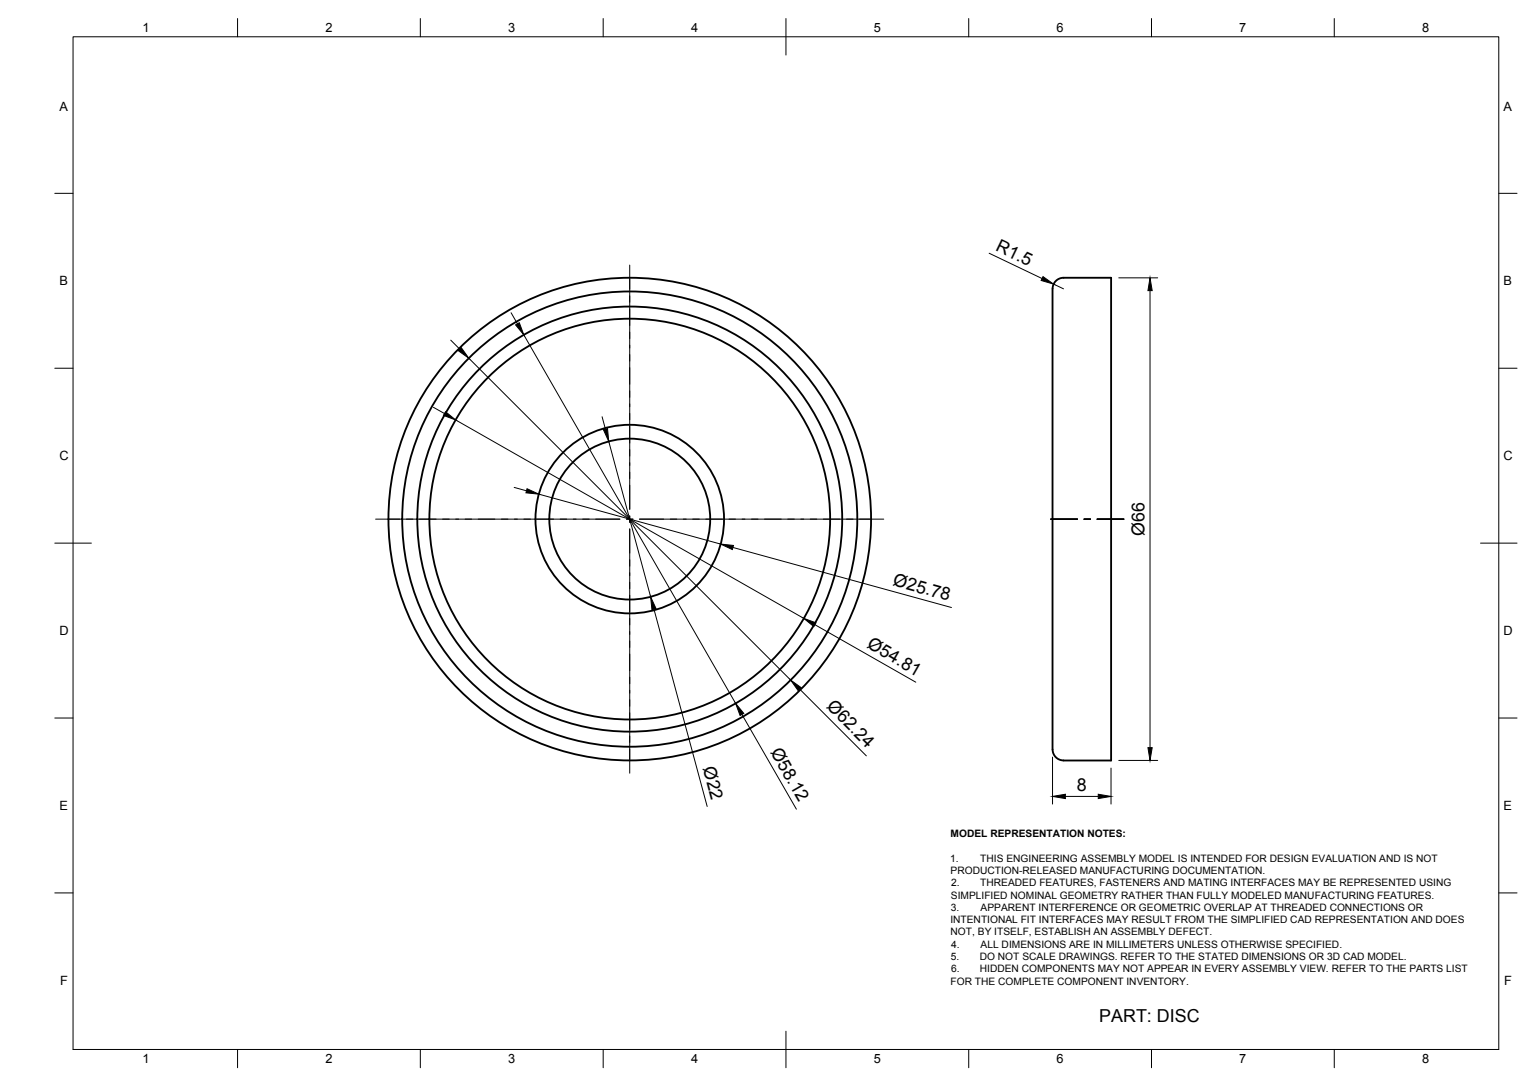
ISO-10303-21;
HEADER;
/* Generated by software containing ST-Developer
 * from STEP Tools, Inc. (www.steptools.com) 
 */

FILE_DESCRIPTION(
/* description */ (''),
/* implementation_level */ '2;1');

FILE_NAME(
/* name */ 'Disc.step',
/* time_stamp */ '2026-10-04T22:47:03-07:00',
/* author */ (''),
/* organization */ (''),
/* preprocessor_version */ 'ST-DEVELOPER v20.2',
/* originating_system */ 'Autodesk Translation Framework v15.15.0.0',
/* authorisation */ '');

FILE_SCHEMA (('AUTOMOTIVE_DESIGN { 1 0 10303 214 3 1 1 }'));
ENDSEC;

DATA;
#10=MECHANICAL_DESIGN_GEOMETRIC_PRESENTATION_REPRESENTATION('',(#81),#19878);
#46=TOROIDAL_SURFACE('',#5269,18.2498324643894,1.5);
#47=TOROIDAL_SURFACE('',#5277,28.1934256722844,1.5);
#48=TOROIDAL_SURFACE('',#5285,31.5,1.5);
#49=TOROIDAL_SURFACE('',#5293,12.,1.);
#67=SHAPE_REPRESENTATION_RELATIONSHIP('SRR','None',#19911,#74);
#74=ADVANCED_BREP_SHAPE_REPRESENTATION('',(#88),#19875);
#81=STYLED_ITEM('',(#19954),#88);
#88=MANIFOLD_SOLID_BREP('Body1',#4829);
#97=FACE_BOUND('',#819,.T.);
#98=FACE_BOUND('',#822,.T.);
#99=FACE_BOUND('',#827,.T.);
#100=FACE_BOUND('',#831,.T.);
#101=FACE_BOUND('',#834,.T.);
#102=FACE_BOUND('',#837,.T.);
#103=FACE_BOUND('',#840,.T.);
#305=PLANE('',#5275);
#306=PLANE('',#5281);
#307=PLANE('',#5290);
#308=PLANE('',#5296);
#309=PLANE('',#5300);
#310=PLANE('',#5304);
#311=PLANE('',#5308);
#534=FACE_OUTER_BOUND('',#816,.T.);
#535=FACE_OUTER_BOUND('',#817,.T.);
#536=FACE_OUTER_BOUND('',#818,.T.);
#537=FACE_OUTER_BOUND('',#820,.T.);
#538=FACE_OUTER_BOUND('',#821,.T.);
#539=FACE_OUTER_BOUND('',#823,.T.);
#540=FACE_OUTER_BOUND('',#824,.T.);
#541=FACE_OUTER_BOUND('',#825,.T.);
#542=FACE_OUTER_BOUND('',#826,.T.);
#543=FACE_OUTER_BOUND('',#828,.T.);
#544=FACE_OUTER_BOUND('',#829,.T.);
#545=FACE_OUTER_BOUND('',#830,.T.);
#546=FACE_OUTER_BOUND('',#832,.T.);
#547=FACE_OUTER_BOUND('',#833,.T.);
#548=FACE_OUTER_BOUND('',#835,.T.);
#549=FACE_OUTER_BOUND('',#836,.T.);
#550=FACE_OUTER_BOUND('',#838,.T.);
#551=FACE_OUTER_BOUND('',#839,.T.);
#816=EDGE_LOOP('',(#4155,#4156,#4157,#4158));
#817=EDGE_LOOP('',(#4159,#4160,#4161,#4162));
#818=EDGE_LOOP('',(#4163));
#819=EDGE_LOOP('',(#4164));
#820=EDGE_LOOP('',(#4165,#4166,#4167,#4168));
#821=EDGE_LOOP('',(#4169));
#822=EDGE_LOOP('',(#4170));
#823=EDGE_LOOP('',(#4171,#4172,#4173,#4174));
#824=EDGE_LOOP('',(#4175,#4176,#4177,#4178));
#825=EDGE_LOOP('',(#4179,#4180,#4181,#4182));
#826=EDGE_LOOP('',(#4183));
#827=EDGE_LOOP('',(#4184));
#828=EDGE_LOOP('',(#4185,#4186,#4187,#4188));
#829=EDGE_LOOP('',(#4189,#4190,#4191,#4192));
#830=EDGE_LOOP('',(#4193));
#831=EDGE_LOOP('',(#4194));
#832=EDGE_LOOP('',(#4195,#4196,#4197,#4198));
#833=EDGE_LOOP('',(#4199));
#834=EDGE_LOOP('',(#4200));
#835=EDGE_LOOP('',(#4201,#4202,#4203,#4204));
#836=EDGE_LOOP('',(#4205));
#837=EDGE_LOOP('',(#4206));
#838=EDGE_LOOP('',(#4207,#4208,#4209,#4210));
#839=EDGE_LOOP('',(#4211));
#840=EDGE_LOOP('',(#4212));
#1197=LINE('',#19572,#1553);
#1198=LINE('',#19589,#1554);
#1199=LINE('',#19596,#1555);
#1200=LINE('',#19602,#1556);
#1201=LINE('',#19613,#1557);
#1202=LINE('',#19620,#1558);
#1203=LINE('',#19627,#1559);
#1553=VECTOR('',#6455,19.7498324643894);
#1554=VECTOR('',#6478,26.6934256722844);
#1555=VECTOR('',#6487,33.);
#1556=VECTOR('',#6496,11.);
#1557=VECTOR('',#6511,27.4027293621977);
#1558=VECTOR('',#6520,29.0578798664922);
#1559=VECTOR('',#6529,31.1192710879259);
#1793=CIRCLE('',#5270,18.2498324643894);
#1794=CIRCLE('',#5271,1.5);
#1795=CIRCLE('',#5272,19.7498324643894);
#1796=CIRCLE('',#5274,19.7498324643894);
#1797=CIRCLE('',#5276,11.);
#1798=CIRCLE('',#5278,26.6934256722844);
#1799=CIRCLE('',#5279,1.5);
#1800=CIRCLE('',#5280,28.1934256722844);
#1801=CIRCLE('',#5282,31.5);
#1802=CIRCLE('',#5284,26.6934256722844);
#1803=CIRCLE('',#5286,1.5);
#1804=CIRCLE('',#5287,33.);
#1805=CIRCLE('',#5289,33.);
#1806=CIRCLE('',#5292,11.);
#1807=CIRCLE('',#5294,12.8892103004758);
#1808=CIRCLE('',#5295,1.);
#1809=CIRCLE('',#5297,27.4027293621977);
#1810=CIRCLE('',#5299,27.4027293621977);
#1811=CIRCLE('',#5301,29.0578798664922);
#1812=CIRCLE('',#5303,29.0578798664922);
#1813=CIRCLE('',#5305,31.1192710879259);
#1814=CIRCLE('',#5307,31.1192710879259);
#2242=VERTEX_POINT('',#19565);
#2243=VERTEX_POINT('',#19567);
#2244=VERTEX_POINT('',#19571);
#2245=VERTEX_POINT('',#19575);
#2246=VERTEX_POINT('',#19578);
#2247=VERTEX_POINT('',#19580);
#2248=VERTEX_POINT('',#19584);
#2249=VERTEX_POINT('',#19587);
#2250=VERTEX_POINT('',#19591);
#2251=VERTEX_POINT('',#19595);
#2252=VERTEX_POINT('',#19600);
#2253=VERTEX_POINT('',#19604);
#2254=VERTEX_POINT('',#19608);
#2255=VERTEX_POINT('',#19611);
#2256=VERTEX_POINT('',#19615);
#2257=VERTEX_POINT('',#19618);
#2258=VERTEX_POINT('',#19622);
#2259=VERTEX_POINT('',#19625);
#2889=EDGE_CURVE('',#2242,#2242,#1793,.T.);
#2890=EDGE_CURVE('',#2242,#2243,#1794,.T.);
#2891=EDGE_CURVE('',#2243,#2243,#1795,.T.);
#2892=EDGE_CURVE('',#2243,#2244,#1197,.T.);
#2893=EDGE_CURVE('',#2244,#2244,#1796,.T.);
#2894=EDGE_CURVE('',#2245,#2245,#1797,.T.);
#2895=EDGE_CURVE('',#2246,#2246,#1798,.T.);
#2896=EDGE_CURVE('',#2246,#2247,#1799,.T.);
#2897=EDGE_CURVE('',#2247,#2247,#1800,.T.);
#2898=EDGE_CURVE('',#2248,#2248,#1801,.T.);
#2899=EDGE_CURVE('',#2249,#2249,#1802,.T.);
#2900=EDGE_CURVE('',#2249,#2246,#1198,.T.);
#2901=EDGE_CURVE('',#2248,#2250,#1803,.T.);
#2902=EDGE_CURVE('',#2250,#2250,#1804,.T.);
#2903=EDGE_CURVE('',#2250,#2251,#1199,.T.);
#2904=EDGE_CURVE('',#2251,#2251,#1805,.T.);
#2905=EDGE_CURVE('',#2252,#2252,#1806,.T.);
#2906=EDGE_CURVE('',#2252,#2245,#1200,.T.);
#2907=EDGE_CURVE('',#2253,#2253,#1807,.T.);
#2908=EDGE_CURVE('',#2253,#2252,#1808,.T.);
#2909=EDGE_CURVE('',#2254,#2254,#1809,.T.);
#2910=EDGE_CURVE('',#2255,#2255,#1810,.T.);
#2911=EDGE_CURVE('',#2255,#2254,#1201,.T.);
#2912=EDGE_CURVE('',#2256,#2256,#1811,.T.);
#2913=EDGE_CURVE('',#2257,#2257,#1812,.T.);
#2914=EDGE_CURVE('',#2257,#2256,#1202,.T.);
#2915=EDGE_CURVE('',#2258,#2258,#1813,.T.);
#2916=EDGE_CURVE('',#2259,#2259,#1814,.T.);
#2917=EDGE_CURVE('',#2259,#2258,#1203,.T.);
#4155=ORIENTED_EDGE('',*,*,#2889,.T.);
#4156=ORIENTED_EDGE('',*,*,#2890,.T.);
#4157=ORIENTED_EDGE('',*,*,#2891,.T.);
#4158=ORIENTED_EDGE('',*,*,#2890,.F.);
#4159=ORIENTED_EDGE('',*,*,#2891,.F.);
#4160=ORIENTED_EDGE('',*,*,#2892,.T.);
#4161=ORIENTED_EDGE('',*,*,#2893,.T.);
#4162=ORIENTED_EDGE('',*,*,#2892,.F.);
#4163=ORIENTED_EDGE('',*,*,#2889,.F.);
#4164=ORIENTED_EDGE('',*,*,#2894,.F.);
#4165=ORIENTED_EDGE('',*,*,#2895,.T.);
#4166=ORIENTED_EDGE('',*,*,#2896,.T.);
#4167=ORIENTED_EDGE('',*,*,#2897,.T.);
#4168=ORIENTED_EDGE('',*,*,#2896,.F.);
#4169=ORIENTED_EDGE('',*,*,#2898,.F.);
#4170=ORIENTED_EDGE('',*,*,#2897,.F.);
#4171=ORIENTED_EDGE('',*,*,#2899,.F.);
#4172=ORIENTED_EDGE('',*,*,#2900,.T.);
#4173=ORIENTED_EDGE('',*,*,#2895,.F.);
#4174=ORIENTED_EDGE('',*,*,#2900,.F.);
#4175=ORIENTED_EDGE('',*,*,#2898,.T.);
#4176=ORIENTED_EDGE('',*,*,#2901,.T.);
#4177=ORIENTED_EDGE('',*,*,#2902,.T.);
#4178=ORIENTED_EDGE('',*,*,#2901,.F.);
#4179=ORIENTED_EDGE('',*,*,#2902,.F.);
#4180=ORIENTED_EDGE('',*,*,#2903,.T.);
#4181=ORIENTED_EDGE('',*,*,#2904,.T.);
#4182=ORIENTED_EDGE('',*,*,#2903,.F.);
#4183=ORIENTED_EDGE('',*,*,#2899,.T.);
#4184=ORIENTED_EDGE('',*,*,#2893,.F.);
#4185=ORIENTED_EDGE('',*,*,#2905,.F.);
#4186=ORIENTED_EDGE('',*,*,#2906,.T.);
#4187=ORIENTED_EDGE('',*,*,#2894,.T.);
#4188=ORIENTED_EDGE('',*,*,#2906,.F.);
#4189=ORIENTED_EDGE('',*,*,#2907,.F.);
#4190=ORIENTED_EDGE('',*,*,#2908,.T.);
#4191=ORIENTED_EDGE('',*,*,#2905,.T.);
#4192=ORIENTED_EDGE('',*,*,#2908,.F.);
#4193=ORIENTED_EDGE('',*,*,#2909,.F.);
#4194=ORIENTED_EDGE('',*,*,#2907,.T.);
#4195=ORIENTED_EDGE('',*,*,#2910,.F.);
#4196=ORIENTED_EDGE('',*,*,#2911,.T.);
#4197=ORIENTED_EDGE('',*,*,#2909,.T.);
#4198=ORIENTED_EDGE('',*,*,#2911,.F.);
#4199=ORIENTED_EDGE('',*,*,#2912,.F.);
#4200=ORIENTED_EDGE('',*,*,#2910,.T.);
#4201=ORIENTED_EDGE('',*,*,#2913,.F.);
#4202=ORIENTED_EDGE('',*,*,#2914,.T.);
#4203=ORIENTED_EDGE('',*,*,#2912,.T.);
#4204=ORIENTED_EDGE('',*,*,#2914,.F.);
#4205=ORIENTED_EDGE('',*,*,#2915,.F.);
#4206=ORIENTED_EDGE('',*,*,#2913,.T.);
#4207=ORIENTED_EDGE('',*,*,#2916,.F.);
#4208=ORIENTED_EDGE('',*,*,#2917,.T.);
#4209=ORIENTED_EDGE('',*,*,#2915,.T.);
#4210=ORIENTED_EDGE('',*,*,#2917,.F.);
#4211=ORIENTED_EDGE('',*,*,#2904,.F.);
#4212=ORIENTED_EDGE('',*,*,#2916,.T.);
#4519=CYLINDRICAL_SURFACE('',#5273,19.7498324643894);
#4520=CYLINDRICAL_SURFACE('',#5283,26.6934256722844);
#4521=CYLINDRICAL_SURFACE('',#5288,33.);
#4522=CYLINDRICAL_SURFACE('',#5291,11.);
#4523=CYLINDRICAL_SURFACE('',#5298,27.4027293621977);
#4524=CYLINDRICAL_SURFACE('',#5302,29.0578798664922);
#4525=CYLINDRICAL_SURFACE('',#5306,31.1192710879259);
#4758=ADVANCED_FACE('',(#534),#46,.T.);
#4759=ADVANCED_FACE('',(#535),#4519,.T.);
#4760=ADVANCED_FACE('',(#536,#97),#305,.T.);
#4761=ADVANCED_FACE('',(#537),#47,.T.);
#4762=ADVANCED_FACE('',(#538,#98),#306,.T.);
#4763=ADVANCED_FACE('',(#539),#4520,.F.);
#4764=ADVANCED_FACE('',(#540),#48,.T.);
#4765=ADVANCED_FACE('',(#541),#4521,.T.);
#4766=ADVANCED_FACE('',(#542,#99),#307,.T.);
#4767=ADVANCED_FACE('',(#543),#4522,.F.);
#4768=ADVANCED_FACE('',(#544),#49,.F.);
#4769=ADVANCED_FACE('',(#545,#100),#308,.T.);
#4770=ADVANCED_FACE('',(#546),#4523,.T.);
#4771=ADVANCED_FACE('',(#547,#101),#309,.T.);
#4772=ADVANCED_FACE('',(#548),#4524,.F.);
#4773=ADVANCED_FACE('',(#549,#102),#310,.T.);
#4774=ADVANCED_FACE('',(#550),#4525,.F.);
#4775=ADVANCED_FACE('',(#551,#103),#311,.T.);
#4829=CLOSED_SHELL('',(#4758,#4759,#4760,#4761,#4762,#4763,#4764,#4765,
#4766,#4767,#4768,#4769,#4770,#4771,#4772,#4773,#4774,#4775));
#5268=AXIS2_PLACEMENT_3D('',#19563,#6443,#6444);
#5269=AXIS2_PLACEMENT_3D('',#19564,#6445,#6446);
#5270=AXIS2_PLACEMENT_3D('',#19566,#6447,#6448);
#5271=AXIS2_PLACEMENT_3D('',#19568,#6449,#6450);
#5272=AXIS2_PLACEMENT_3D('',#19569,#6451,#6452);
#5273=AXIS2_PLACEMENT_3D('',#19570,#6453,#6454);
#5274=AXIS2_PLACEMENT_3D('',#19573,#6456,#6457);
#5275=AXIS2_PLACEMENT_3D('',#19574,#6458,#6459);
#5276=AXIS2_PLACEMENT_3D('',#19576,#6460,#6461);
#5277=AXIS2_PLACEMENT_3D('',#19577,#6462,#6463);
#5278=AXIS2_PLACEMENT_3D('',#19579,#6464,#6465);
#5279=AXIS2_PLACEMENT_3D('',#19581,#6466,#6467);
#5280=AXIS2_PLACEMENT_3D('',#19582,#6468,#6469);
#5281=AXIS2_PLACEMENT_3D('',#19583,#6470,#6471);
#5282=AXIS2_PLACEMENT_3D('',#19585,#6472,#6473);
#5283=AXIS2_PLACEMENT_3D('',#19586,#6474,#6475);
#5284=AXIS2_PLACEMENT_3D('',#19588,#6476,#6477);
#5285=AXIS2_PLACEMENT_3D('',#19590,#6479,#6480);
#5286=AXIS2_PLACEMENT_3D('',#19592,#6481,#6482);
#5287=AXIS2_PLACEMENT_3D('',#19593,#6483,#6484);
#5288=AXIS2_PLACEMENT_3D('',#19594,#6485,#6486);
#5289=AXIS2_PLACEMENT_3D('',#19597,#6488,#6489);
#5290=AXIS2_PLACEMENT_3D('',#19598,#6490,#6491);
#5291=AXIS2_PLACEMENT_3D('',#19599,#6492,#6493);
#5292=AXIS2_PLACEMENT_3D('',#19601,#6494,#6495);
#5293=AXIS2_PLACEMENT_3D('',#19603,#6497,#6498);
#5294=AXIS2_PLACEMENT_3D('',#19605,#6499,#6500);
#5295=AXIS2_PLACEMENT_3D('',#19606,#6501,#6502);
#5296=AXIS2_PLACEMENT_3D('',#19607,#6503,#6504);
#5297=AXIS2_PLACEMENT_3D('',#19609,#6505,#6506);
#5298=AXIS2_PLACEMENT_3D('',#19610,#6507,#6508);
#5299=AXIS2_PLACEMENT_3D('',#19612,#6509,#6510);
#5300=AXIS2_PLACEMENT_3D('',#19614,#6512,#6513);
#5301=AXIS2_PLACEMENT_3D('',#19616,#6514,#6515);
#5302=AXIS2_PLACEMENT_3D('',#19617,#6516,#6517);
#5303=AXIS2_PLACEMENT_3D('',#19619,#6518,#6519);
#5304=AXIS2_PLACEMENT_3D('',#19621,#6521,#6522);
#5305=AXIS2_PLACEMENT_3D('',#19623,#6523,#6524);
#5306=AXIS2_PLACEMENT_3D('',#19624,#6525,#6526);
#5307=AXIS2_PLACEMENT_3D('',#19626,#6527,#6528);
#5308=AXIS2_PLACEMENT_3D('',#19628,#6530,#6531);
#6443=DIRECTION('axis',(0.,0.,1.));
#6444=DIRECTION('refdir',(1.,0.,0.));
#6445=DIRECTION('center_axis',(0.,0.,1.));
#6446=DIRECTION('ref_axis',(1.,0.,0.));
#6447=DIRECTION('center_axis',(0.,0.,-1.));
#6448=DIRECTION('ref_axis',(-1.,1.22464679914735E-16,0.));
#6449=DIRECTION('center_axis',(1.22464679914735E-16,-1.,0.));
#6450=DIRECTION('ref_axis',(-1.,-1.22464679914735E-16,0.));
#6451=DIRECTION('center_axis',(0.,0.,1.));
#6452=DIRECTION('ref_axis',(-1.,1.22464679914735E-16,0.));
#6453=DIRECTION('center_axis',(0.,0.,1.));
#6454=DIRECTION('ref_axis',(1.,0.,0.));
#6455=DIRECTION('',(0.,0.,-1.));
#6456=DIRECTION('center_axis',(0.,0.,1.));
#6457=DIRECTION('ref_axis',(1.,0.,0.));
#6458=DIRECTION('center_axis',(0.,0.,1.));
#6459=DIRECTION('ref_axis',(1.,0.,0.));
#6460=DIRECTION('center_axis',(0.,0.,1.));
#6461=DIRECTION('ref_axis',(1.,0.,0.));
#6462=DIRECTION('center_axis',(0.,0.,1.));
#6463=DIRECTION('ref_axis',(1.,0.,0.));
#6464=DIRECTION('center_axis',(0.,0.,-1.));
#6465=DIRECTION('ref_axis',(-1.,1.22464679914735E-16,0.));
#6466=DIRECTION('center_axis',(1.22464679914735E-16,-1.,0.));
#6467=DIRECTION('ref_axis',(-1.,-1.22464679914735E-16,0.));
#6468=DIRECTION('center_axis',(0.,0.,1.));
#6469=DIRECTION('ref_axis',(-1.,1.22464679914735E-16,0.));
#6470=DIRECTION('center_axis',(0.,0.,1.));
#6471=DIRECTION('ref_axis',(1.,0.,0.));
#6472=DIRECTION('center_axis',(0.,0.,-1.));
#6473=DIRECTION('ref_axis',(-1.,1.22464679914735E-16,0.));
#6474=DIRECTION('center_axis',(0.,0.,1.));
#6475=DIRECTION('ref_axis',(1.,0.,0.));
#6476=DIRECTION('center_axis',(0.,0.,1.));
#6477=DIRECTION('ref_axis',(1.,0.,0.));
#6478=DIRECTION('',(0.,0.,1.));
#6479=DIRECTION('center_axis',(0.,0.,1.));
#6480=DIRECTION('ref_axis',(1.,0.,0.));
#6481=DIRECTION('center_axis',(1.22464679914735E-16,-1.,0.));
#6482=DIRECTION('ref_axis',(-1.,-1.22464679914735E-16,0.));
#6483=DIRECTION('center_axis',(0.,0.,1.));
#6484=DIRECTION('ref_axis',(-1.,1.22464679914735E-16,0.));
#6485=DIRECTION('center_axis',(0.,0.,1.));
#6486=DIRECTION('ref_axis',(1.,0.,0.));
#6487=DIRECTION('',(0.,0.,-1.));
#6488=DIRECTION('center_axis',(0.,0.,1.));
#6489=DIRECTION('ref_axis',(1.,0.,0.));
#6490=DIRECTION('center_axis',(0.,0.,1.));
#6491=DIRECTION('ref_axis',(1.,0.,0.));
#6492=DIRECTION('center_axis',(0.,0.,1.));
#6493=DIRECTION('ref_axis',(1.,0.,0.));
#6494=DIRECTION('center_axis',(0.,0.,1.));
#6495=DIRECTION('ref_axis',(1.,0.,0.));
#6496=DIRECTION('',(0.,0.,1.));
#6497=DIRECTION('center_axis',(0.,0.,1.));
#6498=DIRECTION('ref_axis',(1.,0.,0.));
#6499=DIRECTION('center_axis',(0.,0.,1.));
#6500=DIRECTION('ref_axis',(1.,0.,0.));
#6501=DIRECTION('center_axis',(-1.22464679914735E-16,1.,0.));
#6502=DIRECTION('ref_axis',(-1.,-1.22464679914735E-16,0.));
#6503=DIRECTION('center_axis',(0.,0.,-1.));
#6504=DIRECTION('ref_axis',(-1.,0.,0.));
#6505=DIRECTION('center_axis',(0.,0.,1.));
#6506=DIRECTION('ref_axis',(1.,0.,0.));
#6507=DIRECTION('center_axis',(0.,0.,1.));
#6508=DIRECTION('ref_axis',(1.,0.,0.));
#6509=DIRECTION('center_axis',(0.,0.,1.));
#6510=DIRECTION('ref_axis',(1.,0.,0.));
#6511=DIRECTION('',(0.,0.,-1.));
#6512=DIRECTION('center_axis',(0.,0.,-1.));
#6513=DIRECTION('ref_axis',(-1.,0.,0.));
#6514=DIRECTION('center_axis',(0.,0.,1.));
#6515=DIRECTION('ref_axis',(1.,0.,0.));
#6516=DIRECTION('center_axis',(0.,0.,1.));
#6517=DIRECTION('ref_axis',(1.,0.,0.));
#6518=DIRECTION('center_axis',(0.,0.,1.));
#6519=DIRECTION('ref_axis',(1.,0.,0.));
#6520=DIRECTION('',(0.,0.,1.));
#6521=DIRECTION('center_axis',(0.,0.,-1.));
#6522=DIRECTION('ref_axis',(-1.,0.,0.));
#6523=DIRECTION('center_axis',(0.,0.,1.));
#6524=DIRECTION('ref_axis',(1.,0.,0.));
#6525=DIRECTION('center_axis',(0.,0.,1.));
#6526=DIRECTION('ref_axis',(1.,0.,0.));
#6527=DIRECTION('center_axis',(0.,0.,1.));
#6528=DIRECTION('ref_axis',(1.,0.,0.));
#6529=DIRECTION('',(0.,0.,1.));
#6530=DIRECTION('center_axis',(0.,0.,-1.));
#6531=DIRECTION('ref_axis',(-1.,0.,0.));
#19563=CARTESIAN_POINT('',(0.,0.,0.));
#19564=CARTESIAN_POINT('Origin',(0.,0.,-3.5));
#19565=CARTESIAN_POINT('',(-18.2498324643894,-2.234959891249E-15,-2.));
#19566=CARTESIAN_POINT('Origin',(0.,0.,-2.));
#19567=CARTESIAN_POINT('',(-19.7498324643894,-2.4186569111211E-15,-3.5));
#19568=CARTESIAN_POINT('Origin',(-18.2498324643894,-2.23495989124899E-15,
-3.5));
#19569=CARTESIAN_POINT('Origin',(0.,0.,-3.5));
#19570=CARTESIAN_POINT('Origin',(0.,0.,-2.75451686738248));
#19571=CARTESIAN_POINT('',(-19.7498324643894,-2.4186569111211E-15,-3.50903373476496));
#19572=CARTESIAN_POINT('',(-19.7498324643894,-2.4186569111211E-15,-2.75451686738248));
#19573=CARTESIAN_POINT('Origin',(0.,0.,-3.50903373476496));
#19574=CARTESIAN_POINT('Origin',(11.,0.,-2.));
#19575=CARTESIAN_POINT('',(-11.,-1.34711147906209E-15,-2.));
#19576=CARTESIAN_POINT('Origin',(0.,0.,-2.));
#19577=CARTESIAN_POINT('Origin',(0.,0.,-3.5));
#19578=CARTESIAN_POINT('',(-26.6934256722844,-3.26900183078409E-15,-3.5));
#19579=CARTESIAN_POINT('Origin',(0.,0.,-3.5));
#19580=CARTESIAN_POINT('',(-28.1934256722844,-3.45269885065619E-15,-2.));
#19581=CARTESIAN_POINT('Origin',(-28.1934256722844,-3.45269885065619E-15,
-3.5));
#19582=CARTESIAN_POINT('Origin',(0.,0.,-2.));
#19583=CARTESIAN_POINT('Origin',(26.6934256722844,0.,-2.));
#19584=CARTESIAN_POINT('',(-31.5,-3.85763741731416E-15,-2.));
#19585=CARTESIAN_POINT('Origin',(0.,0.,-2.));
#19586=CARTESIAN_POINT('Origin',(0.,0.,-2.75451686738248));
#19587=CARTESIAN_POINT('',(-26.6934256722844,-3.26900183078409E-15,-3.50903373476496));
#19588=CARTESIAN_POINT('Origin',(0.,0.,-3.50903373476496));
#19589=CARTESIAN_POINT('',(-26.6934256722844,-3.26900183078409E-15,-2.75451686738248));
#19590=CARTESIAN_POINT('Origin',(0.,0.,-3.5));
#19591=CARTESIAN_POINT('',(-33.,-4.04133443718627E-15,-3.5));
#19592=CARTESIAN_POINT('Origin',(-31.5,-3.85763741731416E-15,-3.5));
#19593=CARTESIAN_POINT('Origin',(0.,0.,-3.5));
#19594=CARTESIAN_POINT('Origin',(0.,0.,-6.));
#19595=CARTESIAN_POINT('',(-33.,-4.04133443718627E-15,-10.));
#19596=CARTESIAN_POINT('',(-33.,-4.04133443718627E-15,-6.));
#19597=CARTESIAN_POINT('Origin',(0.,0.,-10.));
#19598=CARTESIAN_POINT('Origin',(19.7498324643894,0.,-3.50903373476496));
#19599=CARTESIAN_POINT('Origin',(0.,0.,-4.36130645705606));
#19600=CARTESIAN_POINT('',(-11.,-1.34711147906209E-15,-6.72261291411212));
#19601=CARTESIAN_POINT('Origin',(0.,0.,-6.72261291411212));
#19602=CARTESIAN_POINT('',(-11.,-1.34711147906209E-15,-4.36130645705606));
#19603=CARTESIAN_POINT('Origin',(0.,0.,-6.72261291411212));
#19604=CARTESIAN_POINT('',(-12.8892103004758,-1.57847301380148E-15,-7.18011159337554));
#19605=CARTESIAN_POINT('Origin',(0.,0.,-7.18011159337554));
#19606=CARTESIAN_POINT('Origin',(-12.,-1.46957615897682E-15,-6.72261291411212));
#19607=CARTESIAN_POINT('Origin',(27.4027293621977,0.,-7.18011159337554));
#19608=CARTESIAN_POINT('',(-27.4027293621977,-3.35586648013166E-15,-7.18011159337554));
#19609=CARTESIAN_POINT('Origin',(0.,0.,-7.18011159337554));
#19610=CARTESIAN_POINT('Origin',(0.,0.,-6.42664169815681));
#19611=CARTESIAN_POINT('',(-27.4027293621977,-3.35586648013166E-15,-5.67317180293808));
#19612=CARTESIAN_POINT('Origin',(0.,0.,-5.67317180293808));
#19613=CARTESIAN_POINT('',(-27.4027293621977,-3.35586648013166E-15,-6.42664169815681));
#19614=CARTESIAN_POINT('Origin',(29.0578798664922,0.,-5.67317180293808));
#19615=CARTESIAN_POINT('',(-29.0578798664922,-3.5585639568508E-15,-5.67317180293808));
#19616=CARTESIAN_POINT('Origin',(0.,0.,-5.67317180293808));
#19617=CARTESIAN_POINT('Origin',(0.,0.,-6.42664169815681));
#19618=CARTESIAN_POINT('',(-29.0578798664922,-3.5585639568508E-15,-7.18011159337554));
#19619=CARTESIAN_POINT('Origin',(0.,0.,-7.18011159337554));
#19620=CARTESIAN_POINT('',(-29.0578798664922,-3.5585639568508E-15,-6.42664169815681));
#19621=CARTESIAN_POINT('Origin',(31.1192710879259,0.,-7.18011159337554));
#19622=CARTESIAN_POINT('',(-31.1192710879259,-3.81101157296272E-15,-7.18011159337554));
#19623=CARTESIAN_POINT('Origin',(0.,0.,-7.18011159337554));
#19624=CARTESIAN_POINT('Origin',(0.,0.,-8.59005579668777));
#19625=CARTESIAN_POINT('',(-31.1192710879259,-3.81101157296272E-15,-10.));
#19626=CARTESIAN_POINT('Origin',(0.,0.,-10.));
#19627=CARTESIAN_POINT('',(-31.1192710879259,-3.81101157296272E-15,-8.59005579668777));
#19628=CARTESIAN_POINT('Origin',(33.,0.,-10.));
#19866=UNCERTAINTY_MEASURE_WITH_UNIT(LENGTH_MEASURE(0.01),#19879,
'DISTANCE_ACCURACY_VALUE',
'Maximum model space distance between geometric entities at asserted c
onnectivities');
#19869=UNCERTAINTY_MEASURE_WITH_UNIT(LENGTH_MEASURE(0.01),#19879,
'DISTANCE_ACCURACY_VALUE',
'Maximum model space distance between geometric entities at asserted c
onnectivities');
#19875=(
GEOMETRIC_REPRESENTATION_CONTEXT(3)
GLOBAL_UNCERTAINTY_ASSIGNED_CONTEXT((#19866))
GLOBAL_UNIT_ASSIGNED_CONTEXT((#19879,#19881,#19882))
REPRESENTATION_CONTEXT('','3D')
);
#19878=(
GEOMETRIC_REPRESENTATION_CONTEXT(3)
GLOBAL_UNCERTAINTY_ASSIGNED_CONTEXT((#19869))
GLOBAL_UNIT_ASSIGNED_CONTEXT((#19879,#19881,#19882))
REPRESENTATION_CONTEXT('','3D')
);
#19879=(
LENGTH_UNIT()
NAMED_UNIT(*)
SI_UNIT(.MILLI.,.METRE.)
);
#19881=(
NAMED_UNIT(*)
PLANE_ANGLE_UNIT()
SI_UNIT($,.RADIAN.)
);
#19882=(
NAMED_UNIT(*)
SI_UNIT($,.STERADIAN.)
SOLID_ANGLE_UNIT()
);
#19888=SHAPE_DEFINITION_REPRESENTATION(#19896,#19911);
#19896=PRODUCT_DEFINITION_SHAPE('',$,#19920);
#19911=SHAPE_REPRESENTATION('',(#5268),#19875);
#19914=PRODUCT_DEFINITION_CONTEXT('part definition',#19940,'design');
#19920=PRODUCT_DEFINITION('Disc','Disc',#19928,#19914);
#19928=PRODUCT_DEFINITION_FORMATION('',$,#19947);
#19940=APPLICATION_CONTEXT(
'Core Data for Automotive Mechanical Design Process');
#19941=PRODUCT_CONTEXT('part definition',#19940,'mechanical');
#19947=PRODUCT('Disc','Disc',$,(#19941));
#19954=PRESENTATION_STYLE_ASSIGNMENT((#19960));
#19960=SURFACE_STYLE_USAGE(.BOTH.,#19966);
#19966=SURFACE_SIDE_STYLE('',(#19972));
#19972=SURFACE_STYLE_FILL_AREA(#19978);
#19978=FILL_AREA_STYLE('Opaque(170,0,255)',(#19984));
#19984=FILL_AREA_STYLE_COLOUR('Opaque(170,0,255)',#19990);
#19990=COLOUR_RGB('Opaque(170,0,255)', 0.72549020, 0.75294118, 0.79215686);
ENDSEC;
END-ISO-10303-21;
